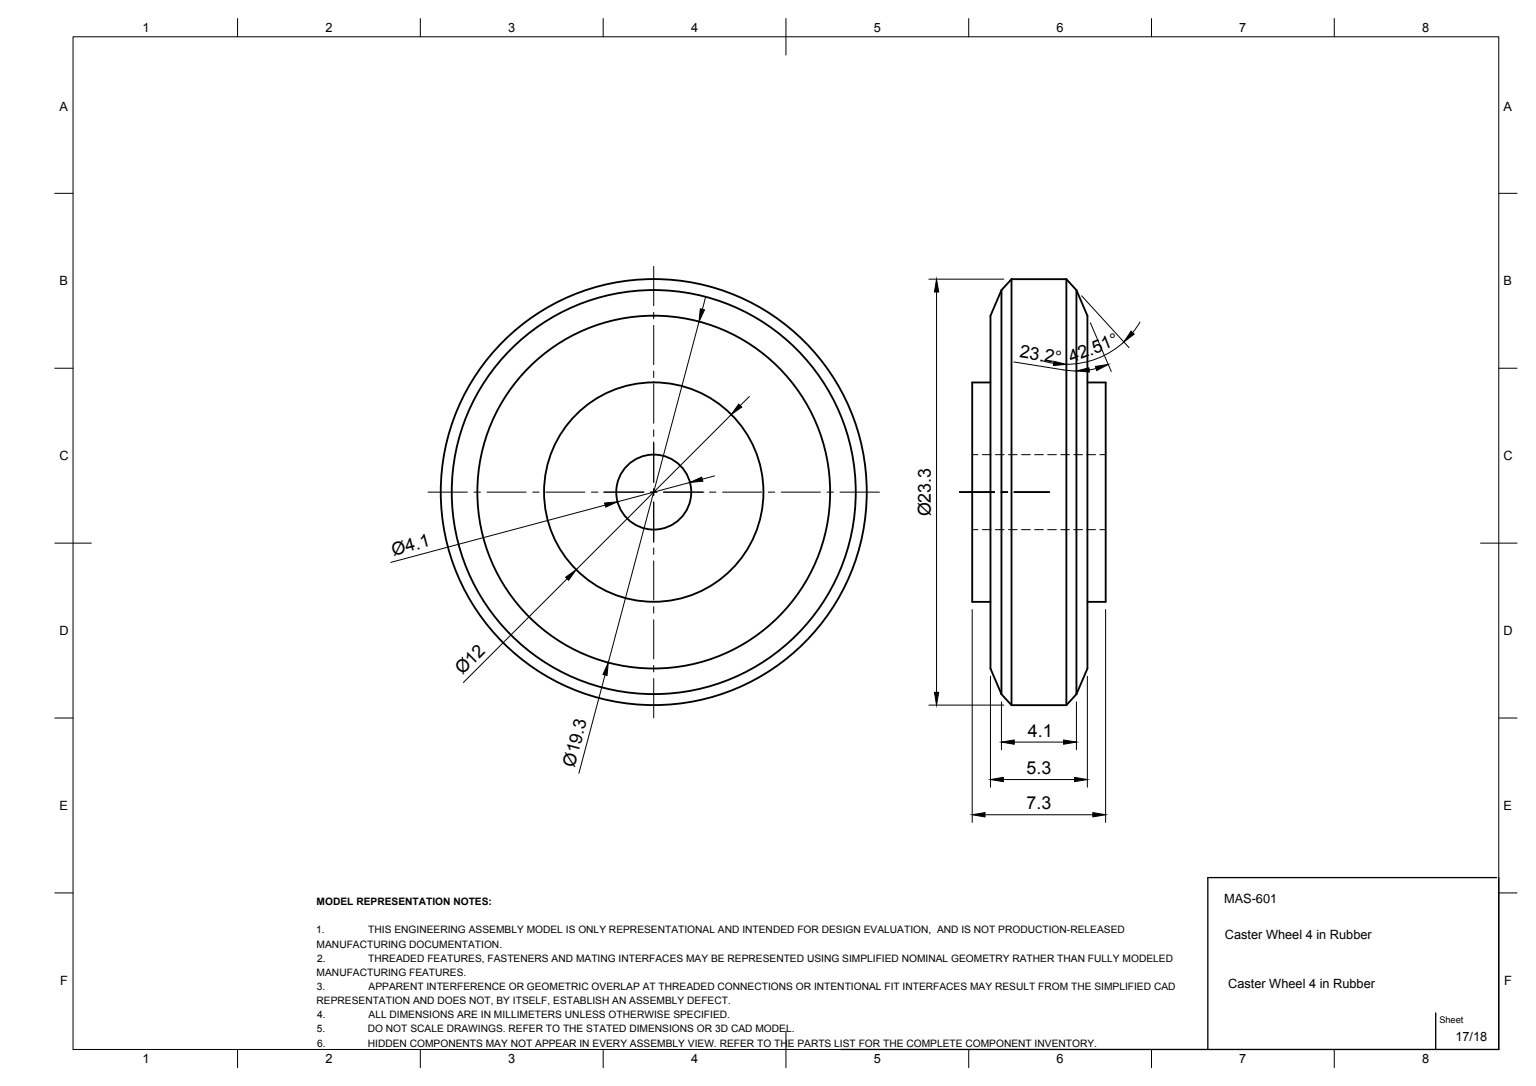
ISO-10303-21;
HEADER;
FILE_DESCRIPTION((''),'2;1');
FILE_NAME('Caster Wheel 4 in Rubber.step','2026-10-06T07:37:42+05:00',(''),(''),'','','');
FILE_SCHEMA (('AUTOMOTIVE_DESIGN { 1 0 10303 214 3 1 1 }'));
ENDSEC;
DATA;
#10=MECHANICAL_DESIGN_GEOMETRIC_PRESENTATION_REPRESENTATION('',(#389),#18757);
#355=SHAPE_REPRESENTATION_RELATIONSHIP('SRR','None',#18873,#372) ;
#372=ADVANCED_BREP_SHAPE_REPRESENTATION('',(#406),#18756) ;
#389=STYLED_ITEM('',(#18967),#406) ;
#406=MANIFOLD_SOLID_BREP('Caster Wheel 4 in Rubber',#9558) ;
#647=CYLINDRICAL_SURFACE('',#10636,6.00000000000001) ;
#648=CYLINDRICAL_SURFACE('',#10644,11.65) ;
#649=CYLINDRICAL_SURFACE('',#10652,6.00000000000001) ;
#650=CYLINDRICAL_SURFACE('',#10656,2.04999999999999) ;
#755=FACE_BOUND('',#2218,.T.) ;
#756=FACE_BOUND('',#2221,.T.) ;
#757=FACE_BOUND('',#2228,.T.) ;
#758=FACE_BOUND('',#2231,.T.) ;
#1083=PLANE('',#10633) ;
#1084=PLANE('',#10638) ;
#1085=PLANE('',#10650) ;
#1086=PLANE('',#10654) ;
#1594=FACE_OUTER_BOUND('',#2217,.T.) ;
#1595=FACE_OUTER_BOUND('',#2219,.T.) ;
#1596=FACE_OUTER_BOUND('',#2220,.T.) ;
#1597=FACE_OUTER_BOUND('',#2222,.T.) ;
#1598=FACE_OUTER_BOUND('',#2223,.T.) ;
#1599=FACE_OUTER_BOUND('',#2224,.T.) ;
#1600=FACE_OUTER_BOUND('',#2225,.T.) ;
#1601=FACE_OUTER_BOUND('',#2226,.T.) ;
#1602=FACE_OUTER_BOUND('',#2227,.T.) ;
#1603=FACE_OUTER_BOUND('',#2229,.T.) ;
#1604=FACE_OUTER_BOUND('',#2230,.T.) ;
#1605=FACE_OUTER_BOUND('',#2232,.T.) ;
#2217=EDGE_LOOP('',(#8953)) ;
#2218=EDGE_LOOP('',(#8954)) ;
#2219=EDGE_LOOP('',(#8955,#8956,#8957,#8958)) ;
#2220=EDGE_LOOP('',(#8959)) ;
#2221=EDGE_LOOP('',(#8960)) ;
#2222=EDGE_LOOP('',(#8961,#8962,#8963,#8964)) ;
#2223=EDGE_LOOP('',(#8965,#8966,#8967,#8968)) ;
#2224=EDGE_LOOP('',(#8969,#8970,#8971,#8972)) ;
#2225=EDGE_LOOP('',(#8973,#8974,#8975,#8976)) ;
#2226=EDGE_LOOP('',(#8977,#8978,#8979,#8980)) ;
#2227=EDGE_LOOP('',(#8981)) ;
#2228=EDGE_LOOP('',(#8982)) ;
#2229=EDGE_LOOP('',(#8983,#8984,#8985,#8986)) ;
#2230=EDGE_LOOP('',(#8987)) ;
#2231=EDGE_LOOP('',(#8988)) ;
#2232=EDGE_LOOP('',(#8989,#8990,#8991,#8992)) ;
#2996=LINE('',#18626,#3767) ;
#2997=LINE('',#18633,#3768) ;
#2998=LINE('',#18637,#3769) ;
#2999=LINE('',#18641,#3770) ;
#3000=LINE('',#18645,#3771) ;
#3001=LINE('',#18649,#3772) ;
#3002=LINE('',#18656,#3773) ;
#3003=LINE('',#18661,#3774) ;
#3767=VECTOR('',#13260,6.00000000000001) ;
#3768=VECTOR('',#13269,10.35) ;
#3769=VECTOR('',#13274,11.35) ;
#3770=VECTOR('',#13279,11.65) ;
#3771=VECTOR('',#13284,11.35) ;
#3772=VECTOR('',#13289,10.35) ;
#3773=VECTOR('',#13298,6.00000000000001) ;
#3774=VECTOR('',#13305,2.04999999999999) ;
#4138=CIRCLE('',#10634,6.00000000000001) ;
#4139=CIRCLE('',#10635,2.04999999999999) ;
#4140=CIRCLE('',#10637,6.00000000000001) ;
#4141=CIRCLE('',#10639,9.65000000000001) ;
#4142=CIRCLE('',#10641,11.05) ;
#4143=CIRCLE('',#10643,11.65) ;
#4144=CIRCLE('',#10645,11.65) ;
#4145=CIRCLE('',#10647,11.05) ;
#4146=CIRCLE('',#10649,9.65000000000001) ;
#4147=CIRCLE('',#10651,6.00000000000001) ;
#4148=CIRCLE('',#10653,6.00000000000001) ;
#4149=CIRCLE('',#10655,2.04999999999999) ;
#5006=VERTEX_POINT('',#18619) ;
#5007=VERTEX_POINT('',#18621) ;
#5008=VERTEX_POINT('',#18624) ;
#5009=VERTEX_POINT('',#18628) ;
#5010=VERTEX_POINT('',#18631) ;
#5011=VERTEX_POINT('',#18635) ;
#5012=VERTEX_POINT('',#18639) ;
#5013=VERTEX_POINT('',#18643) ;
#5014=VERTEX_POINT('',#18647) ;
#5015=VERTEX_POINT('',#18651) ;
#5016=VERTEX_POINT('',#18654) ;
#5017=VERTEX_POINT('',#18658) ;
#6323=EDGE_CURVE('',#5006,#5006,#4138,.T.) ;
#6324=EDGE_CURVE('',#5007,#5007,#4139,.T.) ;
#6325=EDGE_CURVE('',#5008,#5008,#4140,.T.) ;
#6326=EDGE_CURVE('',#5008,#5006,#2996,.T.) ;
#6327=EDGE_CURVE('',#5009,#5009,#4141,.T.) ;
#6328=EDGE_CURVE('',#5010,#5010,#4142,.T.) ;
#6329=EDGE_CURVE('',#5010,#5009,#2997,.T.) ;
#6330=EDGE_CURVE('',#5011,#5011,#4143,.T.) ;
#6331=EDGE_CURVE('',#5011,#5010,#2998,.T.) ;
#6332=EDGE_CURVE('',#5012,#5012,#4144,.T.) ;
#6333=EDGE_CURVE('',#5012,#5011,#2999,.T.) ;
#6334=EDGE_CURVE('',#5013,#5013,#4145,.T.) ;
#6335=EDGE_CURVE('',#5013,#5012,#3000,.T.) ;
#6336=EDGE_CURVE('',#5014,#5014,#4146,.T.) ;
#6337=EDGE_CURVE('',#5014,#5013,#3001,.T.) ;
#6338=EDGE_CURVE('',#5015,#5015,#4147,.T.) ;
#6339=EDGE_CURVE('',#5016,#5016,#4148,.T.) ;
#6340=EDGE_CURVE('',#5016,#5015,#3002,.T.) ;
#6341=EDGE_CURVE('',#5017,#5017,#4149,.T.) ;
#6342=EDGE_CURVE('',#5017,#5007,#3003,.T.) ;
#8953=ORIENTED_EDGE('',*,*,#6323,.F.) ;
#8954=ORIENTED_EDGE('',*,*,#6324,.T.) ;
#8955=ORIENTED_EDGE('',*,*,#6325,.F.) ;
#8956=ORIENTED_EDGE('',*,*,#6326,.T.) ;
#8957=ORIENTED_EDGE('',*,*,#6323,.T.) ;
#8958=ORIENTED_EDGE('',*,*,#6326,.F.) ;
#8959=ORIENTED_EDGE('',*,*,#6327,.F.) ;
#8960=ORIENTED_EDGE('',*,*,#6325,.T.) ;
#8961=ORIENTED_EDGE('',*,*,#6328,.F.) ;
#8962=ORIENTED_EDGE('',*,*,#6329,.T.) ;
#8963=ORIENTED_EDGE('',*,*,#6327,.T.) ;
#8964=ORIENTED_EDGE('',*,*,#6329,.F.) ;
#8965=ORIENTED_EDGE('',*,*,#6330,.F.) ;
#8966=ORIENTED_EDGE('',*,*,#6331,.T.) ;
#8967=ORIENTED_EDGE('',*,*,#6328,.T.) ;
#8968=ORIENTED_EDGE('',*,*,#6331,.F.) ;
#8969=ORIENTED_EDGE('',*,*,#6332,.F.) ;
#8970=ORIENTED_EDGE('',*,*,#6333,.T.) ;
#8971=ORIENTED_EDGE('',*,*,#6330,.T.) ;
#8972=ORIENTED_EDGE('',*,*,#6333,.F.) ;
#8973=ORIENTED_EDGE('',*,*,#6334,.F.) ;
#8974=ORIENTED_EDGE('',*,*,#6335,.T.) ;
#8975=ORIENTED_EDGE('',*,*,#6332,.T.) ;
#8976=ORIENTED_EDGE('',*,*,#6335,.F.) ;
#8977=ORIENTED_EDGE('',*,*,#6336,.F.) ;
#8978=ORIENTED_EDGE('',*,*,#6337,.T.) ;
#8979=ORIENTED_EDGE('',*,*,#6334,.T.) ;
#8980=ORIENTED_EDGE('',*,*,#6337,.F.) ;
#8981=ORIENTED_EDGE('',*,*,#6336,.T.) ;
#8982=ORIENTED_EDGE('',*,*,#6338,.F.) ;
#8983=ORIENTED_EDGE('',*,*,#6339,.F.) ;
#8984=ORIENTED_EDGE('',*,*,#6340,.T.) ;
#8985=ORIENTED_EDGE('',*,*,#6338,.T.) ;
#8986=ORIENTED_EDGE('',*,*,#6340,.F.) ;
#8987=ORIENTED_EDGE('',*,*,#6339,.T.) ;
#8988=ORIENTED_EDGE('',*,*,#6341,.F.) ;
#8989=ORIENTED_EDGE('',*,*,#6341,.T.) ;
#8990=ORIENTED_EDGE('',*,*,#6342,.T.) ;
#8991=ORIENTED_EDGE('',*,*,#6324,.F.) ;
#8992=ORIENTED_EDGE('',*,*,#6342,.F.) ;
#9019=CONICAL_SURFACE('',#10640,10.35,1.16590454050981) ;
#9020=CONICAL_SURFACE('',#10642,11.35,0.828849058788986) ;
#9021=CONICAL_SURFACE('',#10646,11.35,0.828849058788986) ;
#9022=CONICAL_SURFACE('',#10648,10.35,1.16590454050981) ;
#9530=ADVANCED_FACE('',(#1594,#755),#1083,.T.) ;
#9531=ADVANCED_FACE('',(#1595),#647,.T.) ;
#9532=ADVANCED_FACE('',(#1596,#756),#1084,.T.) ;
#9533=ADVANCED_FACE('',(#1597),#9019,.T.) ;
#9534=ADVANCED_FACE('',(#1598),#9020,.T.) ;
#9535=ADVANCED_FACE('',(#1599),#648,.T.) ;
#9536=ADVANCED_FACE('',(#1600),#9021,.T.) ;
#9537=ADVANCED_FACE('',(#1601),#9022,.T.) ;
#9538=ADVANCED_FACE('',(#1602,#757),#1085,.T.) ;
#9539=ADVANCED_FACE('',(#1603),#649,.T.) ;
#9540=ADVANCED_FACE('',(#1604,#758),#1086,.T.) ;
#9541=ADVANCED_FACE('',(#1605),#650,.F.) ;
#9558=CLOSED_SHELL('',(#9530,#9531,#9532,#9533,#9534,#9535,#9536,#9537,
#9538,#9539,#9540,#9541)) ;
#10632=AXIS2_PLACEMENT_3D('',#18617,#13248,#13249) ;
#10633=AXIS2_PLACEMENT_3D('',#18618,#13250,#13251) ;
#10634=AXIS2_PLACEMENT_3D('',#18620,#13252,#13253) ;
#10635=AXIS2_PLACEMENT_3D('',#18622,#13254,#13255) ;
#10636=AXIS2_PLACEMENT_3D('',#18623,#13256,#13257) ;
#10637=AXIS2_PLACEMENT_3D('',#18625,#13258,#13259) ;
#10638=AXIS2_PLACEMENT_3D('',#18627,#13261,#13262) ;
#10639=AXIS2_PLACEMENT_3D('',#18629,#13263,#13264) ;
#10640=AXIS2_PLACEMENT_3D('',#18630,#13265,#13266) ;
#10641=AXIS2_PLACEMENT_3D('',#18632,#13267,#13268) ;
#10642=AXIS2_PLACEMENT_3D('',#18634,#13270,#13271) ;
#10643=AXIS2_PLACEMENT_3D('',#18636,#13272,#13273) ;
#10644=AXIS2_PLACEMENT_3D('',#18638,#13275,#13276) ;
#10645=AXIS2_PLACEMENT_3D('',#18640,#13277,#13278) ;
#10646=AXIS2_PLACEMENT_3D('',#18642,#13280,#13281) ;
#10647=AXIS2_PLACEMENT_3D('',#18644,#13282,#13283) ;
#10648=AXIS2_PLACEMENT_3D('',#18646,#13285,#13286) ;
#10649=AXIS2_PLACEMENT_3D('',#18648,#13287,#13288) ;
#10650=AXIS2_PLACEMENT_3D('',#18650,#13290,#13291) ;
#10651=AXIS2_PLACEMENT_3D('',#18652,#13292,#13293) ;
#10652=AXIS2_PLACEMENT_3D('',#18653,#13294,#13295) ;
#10653=AXIS2_PLACEMENT_3D('',#18655,#13296,#13297) ;
#10654=AXIS2_PLACEMENT_3D('',#18657,#13299,#13300) ;
#10655=AXIS2_PLACEMENT_3D('',#18659,#13301,#13302) ;
#10656=AXIS2_PLACEMENT_3D('',#18660,#13303,#13304) ;
#13248=DIRECTION('axis',(0.,0.,1.)) ;
#13249=DIRECTION('refdir',(1.,0.,0.)) ;
#13250=DIRECTION('center_axis',(0.,1.,0.)) ;
#13251=DIRECTION('ref_axis',(0.,0.,1.)) ;
#13252=DIRECTION('center_axis',(0.,-1.,0.)) ;
#13253=DIRECTION('ref_axis',(1.,0.,0.)) ;
#13254=DIRECTION('center_axis',(0.,-1.,0.)) ;
#13255=DIRECTION('ref_axis',(1.,0.,0.)) ;
#13256=DIRECTION('center_axis',(0.,-1.,0.)) ;
#13257=DIRECTION('ref_axis',(1.,0.,0.)) ;
#13258=DIRECTION('center_axis',(0.,-1.,0.)) ;
#13259=DIRECTION('ref_axis',(1.,0.,0.)) ;
#13260=DIRECTION('',(0.,1.,0.)) ;
#13261=DIRECTION('center_axis',(0.,1.,0.)) ;
#13262=DIRECTION('ref_axis',(0.,0.,1.)) ;
#13263=DIRECTION('center_axis',(0.,-1.,0.)) ;
#13264=DIRECTION('ref_axis',(1.,0.,0.)) ;
#13265=DIRECTION('center_axis',(0.,-1.,0.)) ;
#13266=DIRECTION('ref_axis',(1.,0.,0.)) ;
#13267=DIRECTION('center_axis',(0.,-1.,0.)) ;
#13268=DIRECTION('ref_axis',(1.,0.,0.)) ;
#13269=DIRECTION('',(0.919145030018058,0.393919298579168,1.12562801896381E-16)) ;
#13270=DIRECTION('center_axis',(0.,-1.,0.)) ;
#13271=DIRECTION('ref_axis',(1.,0.,0.)) ;
#13272=DIRECTION('center_axis',(0.,-1.,0.)) ;
#13273=DIRECTION('ref_axis',(1.,0.,0.)) ;
#13274=DIRECTION('',(0.737154140200746,0.675724628517341,9.02753458275063E-17)) ;
#13275=DIRECTION('center_axis',(0.,-1.,0.)) ;
#13276=DIRECTION('ref_axis',(1.,0.,0.)) ;
#13277=DIRECTION('center_axis',(0.,-1.,0.)) ;
#13278=DIRECTION('ref_axis',(1.,0.,0.)) ;
#13279=DIRECTION('',(0.,1.,0.)) ;
#13280=DIRECTION('center_axis',(0.,1.,0.)) ;
#13281=DIRECTION('ref_axis',(1.,0.,0.)) ;
#13282=DIRECTION('center_axis',(0.,-1.,0.)) ;
#13283=DIRECTION('ref_axis',(1.,0.,0.)) ;
#13284=DIRECTION('',(-0.737154140200746,0.675724628517341,-9.02753458275063E-17)) ;
#13285=DIRECTION('center_axis',(0.,1.,0.)) ;
#13286=DIRECTION('ref_axis',(1.,0.,0.)) ;
#13287=DIRECTION('center_axis',(0.,-1.,0.)) ;
#13288=DIRECTION('ref_axis',(1.,0.,0.)) ;
#13289=DIRECTION('',(-0.919145030018055,0.393919298579173,-1.12562801896381E-16)) ;
#13290=DIRECTION('center_axis',(0.,-1.,0.)) ;
#13291=DIRECTION('ref_axis',(0.,0.,-1.)) ;
#13292=DIRECTION('center_axis',(0.,-1.,0.)) ;
#13293=DIRECTION('ref_axis',(1.,0.,0.)) ;
#13294=DIRECTION('center_axis',(0.,-1.,0.)) ;
#13295=DIRECTION('ref_axis',(1.,0.,0.)) ;
#13296=DIRECTION('center_axis',(0.,-1.,0.)) ;
#13297=DIRECTION('ref_axis',(1.,0.,0.)) ;
#13298=DIRECTION('',(0.,1.,0.)) ;
#13299=DIRECTION('center_axis',(0.,-1.,0.)) ;
#13300=DIRECTION('ref_axis',(0.,0.,-1.)) ;
#13301=DIRECTION('center_axis',(0.,-1.,0.)) ;
#13302=DIRECTION('ref_axis',(1.,0.,0.)) ;
#13303=DIRECTION('center_axis',(0.,-1.,0.)) ;
#13304=DIRECTION('ref_axis',(1.,0.,0.)) ;
#13305=DIRECTION('',(0.,1.,0.)) ;
#18617=CARTESIAN_POINT('',(0.,0.,0.)) ;
#18618=CARTESIAN_POINT('Origin',(84.25,55.95,11.65)) ;
#18619=CARTESIAN_POINT('',(72.25,55.95,11.65)) ;
#18620=CARTESIAN_POINT('Origin',(78.25,55.95,11.65)) ;
#18621=CARTESIAN_POINT('',(76.2,55.95,11.65)) ;
#18622=CARTESIAN_POINT('Origin',(78.25,55.95,11.65)) ;
#18623=CARTESIAN_POINT('Origin',(78.25,55.45,11.65)) ;
#18624=CARTESIAN_POINT('',(72.25,54.95,11.65)) ;
#18625=CARTESIAN_POINT('Origin',(78.25,54.95,11.65)) ;
#18626=CARTESIAN_POINT('',(72.25,55.45,11.65)) ;
#18627=CARTESIAN_POINT('Origin',(87.9,54.95,11.65)) ;
#18628=CARTESIAN_POINT('',(68.6,54.95,11.65)) ;
#18629=CARTESIAN_POINT('Origin',(78.25,54.95,11.65)) ;
#18630=CARTESIAN_POINT('Origin',(78.25,54.65,11.65)) ;
#18631=CARTESIAN_POINT('',(67.2,54.35,11.65)) ;
#18632=CARTESIAN_POINT('Origin',(78.25,54.35,11.65)) ;
#18633=CARTESIAN_POINT('',(67.9,54.65,11.65)) ;
#18634=CARTESIAN_POINT('Origin',(78.25,54.075,11.65)) ;
#18635=CARTESIAN_POINT('',(66.6,53.8,11.65)) ;
#18636=CARTESIAN_POINT('Origin',(78.25,53.8,11.65)) ;
#18637=CARTESIAN_POINT('',(66.9,54.075,11.65)) ;
#18638=CARTESIAN_POINT('Origin',(78.25,52.3,11.65)) ;
#18639=CARTESIAN_POINT('',(66.6,50.8,11.65)) ;
#18640=CARTESIAN_POINT('Origin',(78.25,50.8,11.65)) ;
#18641=CARTESIAN_POINT('',(66.6,52.3,11.65)) ;
#18642=CARTESIAN_POINT('Origin',(78.25,50.525,11.65)) ;
#18643=CARTESIAN_POINT('',(67.2,50.25,11.65)) ;
#18644=CARTESIAN_POINT('Origin',(78.25,50.25,11.65)) ;
#18645=CARTESIAN_POINT('',(66.9,50.525,11.65)) ;
#18646=CARTESIAN_POINT('Origin',(78.25,49.95,11.65)) ;
#18647=CARTESIAN_POINT('',(68.6,49.65,11.65)) ;
#18648=CARTESIAN_POINT('Origin',(78.25,49.65,11.65)) ;
#18649=CARTESIAN_POINT('',(67.9,49.95,11.65)) ;
#18650=CARTESIAN_POINT('Origin',(84.25,49.65,11.65)) ;
#18651=CARTESIAN_POINT('',(72.25,49.65,11.65)) ;
#18652=CARTESIAN_POINT('Origin',(78.25,49.65,11.65)) ;
#18653=CARTESIAN_POINT('Origin',(78.25,49.15,11.65)) ;
#18654=CARTESIAN_POINT('',(72.25,48.65,11.65)) ;
#18655=CARTESIAN_POINT('Origin',(78.25,48.65,11.65)) ;
#18656=CARTESIAN_POINT('',(72.25,49.15,11.65)) ;
#18657=CARTESIAN_POINT('Origin',(80.3,48.65,11.65)) ;
#18658=CARTESIAN_POINT('',(76.2,48.65,11.65)) ;
#18659=CARTESIAN_POINT('Origin',(78.25,48.65,11.65)) ;
#18660=CARTESIAN_POINT('Origin',(78.25,52.3,11.65)) ;
#18661=CARTESIAN_POINT('',(76.2,52.3,11.65)) ;
#18737=UNCERTAINTY_MEASURE_WITH_UNIT(LENGTH_MEASURE(0.01),#18758,
'DISTANCE_ACCURACY_VALUE',
'Maximum model space distance between geometric entities at asserted c
onnectivities') ;
#18738=UNCERTAINTY_MEASURE_WITH_UNIT(LENGTH_MEASURE(0.01),#18758,
'DISTANCE_ACCURACY_VALUE',
'Maximum model space distance between geometric entities at asserted c
onnectivities') ;
#18756=(
GEOMETRIC_REPRESENTATION_CONTEXT(3)
GLOBAL_UNCERTAINTY_ASSIGNED_CONTEXT((#18737))
GLOBAL_UNIT_ASSIGNED_CONTEXT((#18758,#18760,#18761))
REPRESENTATION_CONTEXT('','3D')
) ;
#18757=(
GEOMETRIC_REPRESENTATION_CONTEXT(3)
GLOBAL_UNCERTAINTY_ASSIGNED_CONTEXT((#18738))
GLOBAL_UNIT_ASSIGNED_CONTEXT((#18758,#18760,#18761))
REPRESENTATION_CONTEXT('','3D')
) ;
#18758=(
LENGTH_UNIT()
NAMED_UNIT(*)
SI_UNIT(.MILLI.,.METRE.)
) ;
#18760=(
NAMED_UNIT(*)
PLANE_ANGLE_UNIT()
SI_UNIT($,.RADIAN.)
) ;
#18761=(
NAMED_UNIT(*)
SI_UNIT($,.STERADIAN.)
SOLID_ANGLE_UNIT()
) ;
#18779=SHAPE_DEFINITION_REPRESENTATION(#18797,#18873) ;
#18797=PRODUCT_DEFINITION_SHAPE('',$,#18892) ;
#18873=SHAPE_REPRESENTATION('',(#10632),#18756) ;
#18874=PRODUCT_DEFINITION_CONTEXT('part definition',#18930,'design') ;
#18892=PRODUCT_DEFINITION('Caster Wheel 4 in Rubber',
'Caster Wheel 4 in Rubber',#18910,#18874) ;
#18910=PRODUCT_DEFINITION_FORMATION('',$,#18949) ;
#18930=APPLICATION_CONTEXT(
'Core Data for Automotive Mechanical Design Process') ;
#18931=PRODUCT_CONTEXT('part definition',#18930,'mechanical') ;
#18949=PRODUCT('Caster Wheel 4 in Rubber','Caster Wheel 4 in Rubber',$,(#18931)) ;
#18967=PRESENTATION_STYLE_ASSIGNMENT((#18985)) ;
#18985=SURFACE_STYLE_USAGE(.BOTH.,#19003) ;
#19003=SURFACE_SIDE_STYLE('',(#19021)) ;
#19021=SURFACE_STYLE_FILL_AREA(#19039) ;
#19039=FILL_AREA_STYLE(
'MAS-253 Metallic Sheet - Caster Wheel 4 in Rubber',(#19057)) ;
#19057=FILL_AREA_STYLE_COLOUR(
'MAS-253 Metallic Sheet - Caster Wheel 4 in Rubber',#19075) ;
#19075=COLOUR_RGB('MAS-253 Metallic Sheet - Caster Wheel 4 in Rubber', 0.08235294, 0.09019608, 0.10196078) ;
ENDSEC;
END-ISO-10303-21;
